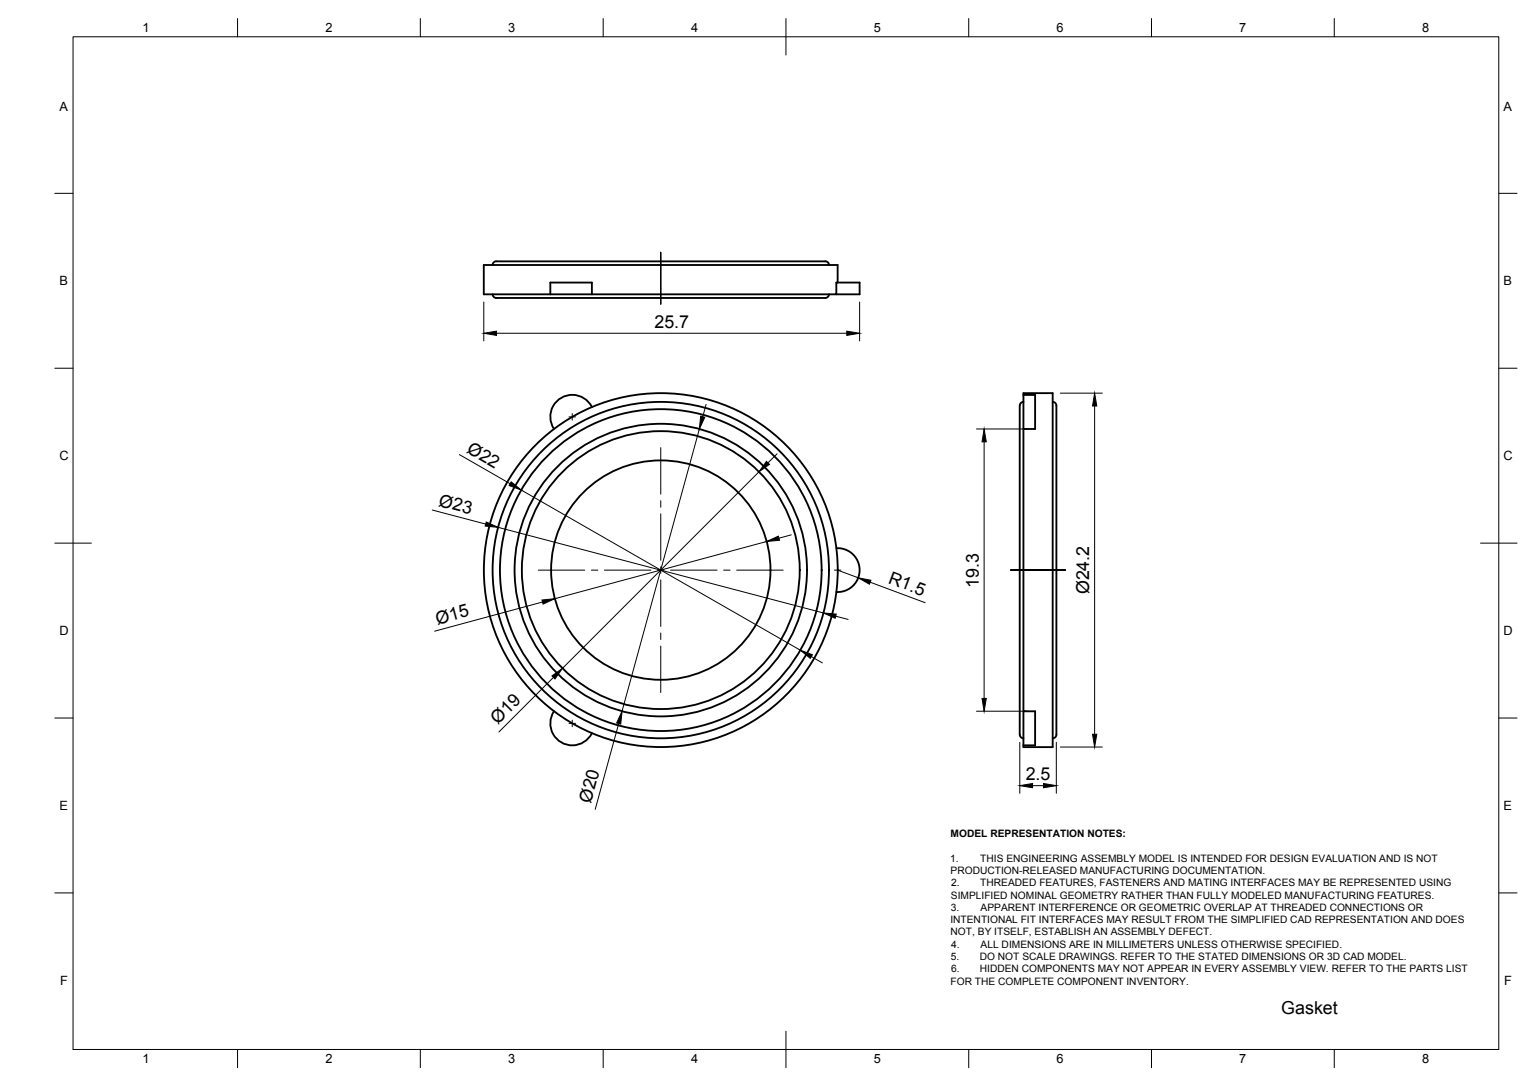
ISO-10303-21;
HEADER;
/* Generated by software containing ST-Developer
 * from STEP Tools, Inc. (www.steptools.com) 
 */

FILE_DESCRIPTION(
/* description */ ('STEP AP214'),
/* implementation_level */ '2;1');

FILE_NAME(
/* name */ 'Gasket.step',
/* time_stamp */ '2026-10-05T23:18:41-07:00',
/* author */ (''),
/* organization */ (''),
/* preprocessor_version */ 'ST-DEVELOPER v20.2',
/* originating_system */ 'Autodesk Translation Framework v15.15.0.0',
/* authorisation */ '');

FILE_SCHEMA (('AUTOMOTIVE_DESIGN { 1 0 10303 214 3 1 1 }'));
ENDSEC;

DATA;
#10=MECHANICAL_DESIGN_GEOMETRIC_PRESENTATION_REPRESENTATION('',(#105),#221662);
#67=MANIFOLD_SOLID_BREP('Body1',#79327);
#79=SHAPE_REPRESENTATION_RELATIONSHIP('SRR','None',#221714,#92);
#92=ADVANCED_BREP_SHAPE_REPRESENTATION('',(#67),#221654);
#105=STYLED_ITEM('',(#221783),#67);
#291=FACE_BOUND('',#24797,.T.);
#292=FACE_BOUND('',#24799,.T.);
#293=FACE_BOUND('',#24801,.T.);
#294=FACE_BOUND('',#24803,.T.);
#295=FACE_BOUND('',#24805,.T.);
#296=FACE_BOUND('',#24807,.T.);
#1892=TOROIDAL_SURFACE('',#80720,9.75,0.25);
#1893=TOROIDAL_SURFACE('',#80724,11.25,0.25);
#1894=TOROIDAL_SURFACE('',#80737,11.25,0.25);
#1895=TOROIDAL_SURFACE('',#80741,9.75,0.25);
#2228=CYLINDRICAL_SURFACE('',#80728,12.1);
#2229=CYLINDRICAL_SURFACE('',#80745,7.50000000000001);
#2230=CYLINDRICAL_SURFACE('',#80748,1.5);
#2231=CYLINDRICAL_SURFACE('',#80751,1.5);
#2232=CYLINDRICAL_SURFACE('',#80757,1.5);
#3145=LINE('',#177883,#10212);
#3146=LINE('',#177887,#10213);
#3147=LINE('',#177891,#10214);
#3148=LINE('',#177895,#10215);
#3149=LINE('',#177899,#10216);
#3150=LINE('',#177903,#10217);
#3151=LINE('',#177907,#10218);
#3152=LINE('',#177925,#10219);
#10212=VECTOR('',#89104,12.1);
#10213=VECTOR('',#89107,1000.);
#10214=VECTOR('',#89110,1000.);
#10215=VECTOR('',#89113,1000.);
#10216=VECTOR('',#89116,1000.);
#10217=VECTOR('',#89119,1000.);
#10218=VECTOR('',#89122,1000.);
#10219=VECTOR('',#89145,7.50000000000001);
#16980=PLANE('',#80754);
#16981=PLANE('',#80755);
#16982=PLANE('',#80759);
#16983=PLANE('',#80760);
#16984=PLANE('',#80761);
#16985=PLANE('',#80762);
#16986=PLANE('',#80763);
#16987=PLANE('',#80764);
#16988=PLANE('',#80765);
#20723=FACE_OUTER_BOUND('',#24784,.T.);
#20724=FACE_OUTER_BOUND('',#24785,.T.);
#20725=FACE_OUTER_BOUND('',#24786,.T.);
#20726=FACE_OUTER_BOUND('',#24787,.T.);
#20727=FACE_OUTER_BOUND('',#24788,.T.);
#20728=FACE_OUTER_BOUND('',#24789,.T.);
#20729=FACE_OUTER_BOUND('',#24790,.T.);
#20730=FACE_OUTER_BOUND('',#24791,.T.);
#20731=FACE_OUTER_BOUND('',#24792,.T.);
#20732=FACE_OUTER_BOUND('',#24793,.T.);
#20733=FACE_OUTER_BOUND('',#24794,.T.);
#20734=FACE_OUTER_BOUND('',#24795,.T.);
#20735=FACE_OUTER_BOUND('',#24796,.T.);
#20736=FACE_OUTER_BOUND('',#24798,.T.);
#20737=FACE_OUTER_BOUND('',#24800,.T.);
#20738=FACE_OUTER_BOUND('',#24802,.T.);
#20739=FACE_OUTER_BOUND('',#24804,.T.);
#20740=FACE_OUTER_BOUND('',#24806,.T.);
#24784=EDGE_LOOP('',(#56581,#56582,#56583,#56584));
#24785=EDGE_LOOP('',(#56585,#56586,#56587,#56588));
#24786=EDGE_LOOP('',(#56589,#56590,#56591,#56592,#56593,#56594,#56595,#56596,
#56597,#56598,#56599,#56600,#56601,#56602,#56603,#56604));
#24787=EDGE_LOOP('',(#56605,#56606,#56607,#56608));
#24788=EDGE_LOOP('',(#56609,#56610,#56611,#56612));
#24789=EDGE_LOOP('',(#56613,#56614,#56615,#56616));
#24790=EDGE_LOOP('',(#56617,#56618,#56619,#56620));
#24791=EDGE_LOOP('',(#56621,#56622,#56623,#56624));
#24792=EDGE_LOOP('',(#56625,#56626));
#24793=EDGE_LOOP('',(#56627,#56628));
#24794=EDGE_LOOP('',(#56629,#56630,#56631,#56632));
#24795=EDGE_LOOP('',(#56633,#56634));
#24796=EDGE_LOOP('',(#56635));
#24797=EDGE_LOOP('',(#56636));
#24798=EDGE_LOOP('',(#56637));
#24799=EDGE_LOOP('',(#56638));
#24800=EDGE_LOOP('',(#56639));
#24801=EDGE_LOOP('',(#56640));
#24802=EDGE_LOOP('',(#56641,#56642,#56643,#56644,#56645,#56646,#56647));
#24803=EDGE_LOOP('',(#56648));
#24804=EDGE_LOOP('',(#56649));
#24805=EDGE_LOOP('',(#56650));
#24806=EDGE_LOOP('',(#56651));
#24807=EDGE_LOOP('',(#56652));
#31271=CIRCLE('',#80721,9.49999999999999);
#31272=CIRCLE('',#80722,0.25);
#31273=CIRCLE('',#80723,10.);
#31274=CIRCLE('',#80725,11.);
#31275=CIRCLE('',#80726,0.25);
#31276=CIRCLE('',#80727,11.5);
#31277=CIRCLE('',#80729,12.1);
#31278=CIRCLE('',#80730,12.1);
#31279=CIRCLE('',#80731,12.1);
#31280=CIRCLE('',#80732,12.1);
#31281=CIRCLE('',#80733,12.1);
#31282=CIRCLE('',#80734,12.1);
#31283=CIRCLE('',#80735,12.1);
#31284=CIRCLE('',#80736,12.1);
#31285=CIRCLE('',#80738,11.5);
#31286=CIRCLE('',#80739,0.25);
#31287=CIRCLE('',#80740,11.);
#31288=CIRCLE('',#80742,10.);
#31289=CIRCLE('',#80743,0.25);
#31290=CIRCLE('',#80744,9.49999999999999);
#31291=CIRCLE('',#80746,7.50000000000001);
#31292=CIRCLE('',#80747,7.50000000000001);
#31293=CIRCLE('',#80749,1.5);
#31294=CIRCLE('',#80750,1.5);
#31295=CIRCLE('',#80752,1.49999999999999);
#31296=CIRCLE('',#80753,1.49999999999999);
#31297=CIRCLE('',#80756,1.5);
#31298=CIRCLE('',#80758,1.5);
#34834=VERTEX_POINT('',#177868);
#34835=VERTEX_POINT('',#177870);
#34836=VERTEX_POINT('',#177874);
#34837=VERTEX_POINT('',#177876);
#34838=VERTEX_POINT('',#177880);
#34839=VERTEX_POINT('',#177882);
#34840=VERTEX_POINT('',#177884);
#34841=VERTEX_POINT('',#177886);
#34842=VERTEX_POINT('',#177888);
#34843=VERTEX_POINT('',#177890);
#34844=VERTEX_POINT('',#177892);
#34845=VERTEX_POINT('',#177894);
#34846=VERTEX_POINT('',#177896);
#34847=VERTEX_POINT('',#177898);
#34848=VERTEX_POINT('',#177900);
#34849=VERTEX_POINT('',#177902);
#34850=VERTEX_POINT('',#177904);
#34851=VERTEX_POINT('',#177906);
#34852=VERTEX_POINT('',#177910);
#34853=VERTEX_POINT('',#177912);
#34854=VERTEX_POINT('',#177916);
#34855=VERTEX_POINT('',#177918);
#34856=VERTEX_POINT('',#177922);
#34857=VERTEX_POINT('',#177924);
#43123=EDGE_CURVE('',#34834,#34834,#31271,.T.);
#43124=EDGE_CURVE('',#34834,#34835,#31272,.T.);
#43125=EDGE_CURVE('',#34835,#34835,#31273,.T.);
#43126=EDGE_CURVE('',#34836,#34836,#31274,.T.);
#43127=EDGE_CURVE('',#34836,#34837,#31275,.T.);
#43128=EDGE_CURVE('',#34837,#34837,#31276,.T.);
#43129=EDGE_CURVE('',#34838,#34838,#31277,.T.);
#43130=EDGE_CURVE('',#34838,#34839,#3145,.T.);
#43131=EDGE_CURVE('',#34839,#34840,#31278,.T.);
#43132=EDGE_CURVE('',#34841,#34840,#3146,.T.);
#43133=EDGE_CURVE('',#34841,#34842,#31279,.T.);
#43134=EDGE_CURVE('',#34843,#34842,#3147,.T.);
#43135=EDGE_CURVE('',#34843,#34844,#31280,.T.);
#43136=EDGE_CURVE('',#34845,#34844,#3148,.T.);
#43137=EDGE_CURVE('',#34845,#34846,#31281,.T.);
#43138=EDGE_CURVE('',#34847,#34846,#3149,.T.);
#43139=EDGE_CURVE('',#34847,#34848,#31282,.T.);
#43140=EDGE_CURVE('',#34849,#34848,#3150,.T.);
#43141=EDGE_CURVE('',#34849,#34850,#31283,.T.);
#43142=EDGE_CURVE('',#34851,#34850,#3151,.T.);
#43143=EDGE_CURVE('',#34851,#34839,#31284,.T.);
#43144=EDGE_CURVE('',#34852,#34852,#31285,.T.);
#43145=EDGE_CURVE('',#34852,#34853,#31286,.T.);
#43146=EDGE_CURVE('',#34853,#34853,#31287,.T.);
#43147=EDGE_CURVE('',#34854,#34854,#31288,.T.);
#43148=EDGE_CURVE('',#34854,#34855,#31289,.T.);
#43149=EDGE_CURVE('',#34855,#34855,#31290,.T.);
#43150=EDGE_CURVE('',#34856,#34856,#31291,.T.);
#43151=EDGE_CURVE('',#34856,#34857,#3152,.T.);
#43152=EDGE_CURVE('',#34857,#34857,#31292,.T.);
#43153=EDGE_CURVE('',#34850,#34849,#31293,.T.);
#43154=EDGE_CURVE('',#34851,#34848,#31294,.T.);
#43155=EDGE_CURVE('',#34842,#34841,#31295,.T.);
#43156=EDGE_CURVE('',#34843,#34840,#31296,.T.);
#43157=EDGE_CURVE('',#34846,#34845,#31297,.T.);
#43158=EDGE_CURVE('',#34847,#34844,#31298,.T.);
#56581=ORIENTED_EDGE('',*,*,#43123,.F.);
#56582=ORIENTED_EDGE('',*,*,#43124,.T.);
#56583=ORIENTED_EDGE('',*,*,#43125,.T.);
#56584=ORIENTED_EDGE('',*,*,#43124,.F.);
#56585=ORIENTED_EDGE('',*,*,#43126,.F.);
#56586=ORIENTED_EDGE('',*,*,#43127,.T.);
#56587=ORIENTED_EDGE('',*,*,#43128,.T.);
#56588=ORIENTED_EDGE('',*,*,#43127,.F.);
#56589=ORIENTED_EDGE('',*,*,#43129,.F.);
#56590=ORIENTED_EDGE('',*,*,#43130,.T.);
#56591=ORIENTED_EDGE('',*,*,#43131,.T.);
#56592=ORIENTED_EDGE('',*,*,#43132,.F.);
#56593=ORIENTED_EDGE('',*,*,#43133,.T.);
#56594=ORIENTED_EDGE('',*,*,#43134,.F.);
#56595=ORIENTED_EDGE('',*,*,#43135,.T.);
#56596=ORIENTED_EDGE('',*,*,#43136,.F.);
#56597=ORIENTED_EDGE('',*,*,#43137,.T.);
#56598=ORIENTED_EDGE('',*,*,#43138,.F.);
#56599=ORIENTED_EDGE('',*,*,#43139,.T.);
#56600=ORIENTED_EDGE('',*,*,#43140,.F.);
#56601=ORIENTED_EDGE('',*,*,#43141,.T.);
#56602=ORIENTED_EDGE('',*,*,#43142,.F.);
#56603=ORIENTED_EDGE('',*,*,#43143,.T.);
#56604=ORIENTED_EDGE('',*,*,#43130,.F.);
#56605=ORIENTED_EDGE('',*,*,#43144,.F.);
#56606=ORIENTED_EDGE('',*,*,#43145,.T.);
#56607=ORIENTED_EDGE('',*,*,#43146,.T.);
#56608=ORIENTED_EDGE('',*,*,#43145,.F.);
#56609=ORIENTED_EDGE('',*,*,#43147,.F.);
#56610=ORIENTED_EDGE('',*,*,#43148,.T.);
#56611=ORIENTED_EDGE('',*,*,#43149,.T.);
#56612=ORIENTED_EDGE('',*,*,#43148,.F.);
#56613=ORIENTED_EDGE('',*,*,#43150,.F.);
#56614=ORIENTED_EDGE('',*,*,#43151,.T.);
#56615=ORIENTED_EDGE('',*,*,#43152,.T.);
#56616=ORIENTED_EDGE('',*,*,#43151,.F.);
#56617=ORIENTED_EDGE('',*,*,#43153,.T.);
#56618=ORIENTED_EDGE('',*,*,#43140,.T.);
#56619=ORIENTED_EDGE('',*,*,#43154,.F.);
#56620=ORIENTED_EDGE('',*,*,#43142,.T.);
#56621=ORIENTED_EDGE('',*,*,#43155,.T.);
#56622=ORIENTED_EDGE('',*,*,#43132,.T.);
#56623=ORIENTED_EDGE('',*,*,#43156,.F.);
#56624=ORIENTED_EDGE('',*,*,#43134,.T.);
#56625=ORIENTED_EDGE('',*,*,#43133,.F.);
#56626=ORIENTED_EDGE('',*,*,#43155,.F.);
#56627=ORIENTED_EDGE('',*,*,#43137,.F.);
#56628=ORIENTED_EDGE('',*,*,#43157,.F.);
#56629=ORIENTED_EDGE('',*,*,#43158,.F.);
#56630=ORIENTED_EDGE('',*,*,#43138,.T.);
#56631=ORIENTED_EDGE('',*,*,#43157,.T.);
#56632=ORIENTED_EDGE('',*,*,#43136,.T.);
#56633=ORIENTED_EDGE('',*,*,#43141,.F.);
#56634=ORIENTED_EDGE('',*,*,#43153,.F.);
#56635=ORIENTED_EDGE('',*,*,#43123,.T.);
#56636=ORIENTED_EDGE('',*,*,#43152,.F.);
#56637=ORIENTED_EDGE('',*,*,#43149,.F.);
#56638=ORIENTED_EDGE('',*,*,#43150,.T.);
#56639=ORIENTED_EDGE('',*,*,#43146,.F.);
#56640=ORIENTED_EDGE('',*,*,#43147,.T.);
#56641=ORIENTED_EDGE('',*,*,#43135,.F.);
#56642=ORIENTED_EDGE('',*,*,#43156,.T.);
#56643=ORIENTED_EDGE('',*,*,#43131,.F.);
#56644=ORIENTED_EDGE('',*,*,#43143,.F.);
#56645=ORIENTED_EDGE('',*,*,#43154,.T.);
#56646=ORIENTED_EDGE('',*,*,#43139,.F.);
#56647=ORIENTED_EDGE('',*,*,#43158,.T.);
#56648=ORIENTED_EDGE('',*,*,#43144,.T.);
#56649=ORIENTED_EDGE('',*,*,#43129,.T.);
#56650=ORIENTED_EDGE('',*,*,#43128,.F.);
#56651=ORIENTED_EDGE('',*,*,#43126,.T.);
#56652=ORIENTED_EDGE('',*,*,#43125,.F.);
#76153=ADVANCED_FACE('',(#20723),#1892,.T.);
#76154=ADVANCED_FACE('',(#20724),#1893,.T.);
#76155=ADVANCED_FACE('',(#20725),#2228,.T.);
#76156=ADVANCED_FACE('',(#20726),#1894,.T.);
#76157=ADVANCED_FACE('',(#20727),#1895,.T.);
#76158=ADVANCED_FACE('',(#20728),#2229,.F.);
#76159=ADVANCED_FACE('',(#20729),#2230,.T.);
#76160=ADVANCED_FACE('',(#20730),#2231,.T.);
#76161=ADVANCED_FACE('',(#20731),#16980,.F.);
#76162=ADVANCED_FACE('',(#20732),#16981,.F.);
#76163=ADVANCED_FACE('',(#20733),#2232,.T.);
#76164=ADVANCED_FACE('',(#20734),#16982,.F.);
#76165=ADVANCED_FACE('',(#20735,#291),#16983,.T.);
#76166=ADVANCED_FACE('',(#20736,#292),#16984,.T.);
#76167=ADVANCED_FACE('',(#20737,#293),#16985,.T.);
#76168=ADVANCED_FACE('',(#20738,#294),#16986,.T.);
#76169=ADVANCED_FACE('',(#20739,#295),#16987,.T.);
#76170=ADVANCED_FACE('',(#20740,#296),#16988,.T.);
#79327=CLOSED_SHELL('',(#76153,#76154,#76155,#76156,#76157,#76158,#76159,
#76160,#76161,#76162,#76163,#76164,#76165,#76166,#76167,#76168,#76169,#76170));
#80719=AXIS2_PLACEMENT_3D('',#177866,#89082,#89083);
#80720=AXIS2_PLACEMENT_3D('',#177867,#89084,#89085);
#80721=AXIS2_PLACEMENT_3D('',#177869,#89086,#89087);
#80722=AXIS2_PLACEMENT_3D('',#177871,#89088,#89089);
#80723=AXIS2_PLACEMENT_3D('',#177872,#89090,#89091);
#80724=AXIS2_PLACEMENT_3D('',#177873,#89092,#89093);
#80725=AXIS2_PLACEMENT_3D('',#177875,#89094,#89095);
#80726=AXIS2_PLACEMENT_3D('',#177877,#89096,#89097);
#80727=AXIS2_PLACEMENT_3D('',#177878,#89098,#89099);
#80728=AXIS2_PLACEMENT_3D('',#177879,#89100,#89101);
#80729=AXIS2_PLACEMENT_3D('',#177881,#89102,#89103);
#80730=AXIS2_PLACEMENT_3D('',#177885,#89105,#89106);
#80731=AXIS2_PLACEMENT_3D('',#177889,#89108,#89109);
#80732=AXIS2_PLACEMENT_3D('',#177893,#89111,#89112);
#80733=AXIS2_PLACEMENT_3D('',#177897,#89114,#89115);
#80734=AXIS2_PLACEMENT_3D('',#177901,#89117,#89118);
#80735=AXIS2_PLACEMENT_3D('',#177905,#89120,#89121);
#80736=AXIS2_PLACEMENT_3D('',#177908,#89123,#89124);
#80737=AXIS2_PLACEMENT_3D('',#177909,#89125,#89126);
#80738=AXIS2_PLACEMENT_3D('',#177911,#89127,#89128);
#80739=AXIS2_PLACEMENT_3D('',#177913,#89129,#89130);
#80740=AXIS2_PLACEMENT_3D('',#177914,#89131,#89132);
#80741=AXIS2_PLACEMENT_3D('',#177915,#89133,#89134);
#80742=AXIS2_PLACEMENT_3D('',#177917,#89135,#89136);
#80743=AXIS2_PLACEMENT_3D('',#177919,#89137,#89138);
#80744=AXIS2_PLACEMENT_3D('',#177920,#89139,#89140);
#80745=AXIS2_PLACEMENT_3D('',#177921,#89141,#89142);
#80746=AXIS2_PLACEMENT_3D('',#177923,#89143,#89144);
#80747=AXIS2_PLACEMENT_3D('',#177926,#89146,#89147);
#80748=AXIS2_PLACEMENT_3D('',#177927,#89148,#89149);
#80749=AXIS2_PLACEMENT_3D('',#177928,#89150,#89151);
#80750=AXIS2_PLACEMENT_3D('',#177929,#89152,#89153);
#80751=AXIS2_PLACEMENT_3D('',#177930,#89154,#89155);
#80752=AXIS2_PLACEMENT_3D('',#177931,#89156,#89157);
#80753=AXIS2_PLACEMENT_3D('',#177932,#89158,#89159);
#80754=AXIS2_PLACEMENT_3D('',#177933,#89160,#89161);
#80755=AXIS2_PLACEMENT_3D('',#177934,#89162,#89163);
#80756=AXIS2_PLACEMENT_3D('',#177935,#89164,#89165);
#80757=AXIS2_PLACEMENT_3D('',#177936,#89166,#89167);
#80758=AXIS2_PLACEMENT_3D('',#177937,#89168,#89169);
#80759=AXIS2_PLACEMENT_3D('',#177938,#89170,#89171);
#80760=AXIS2_PLACEMENT_3D('',#177939,#89172,#89173);
#80761=AXIS2_PLACEMENT_3D('',#177940,#89174,#89175);
#80762=AXIS2_PLACEMENT_3D('',#177941,#89176,#89177);
#80763=AXIS2_PLACEMENT_3D('',#177942,#89178,#89179);
#80764=AXIS2_PLACEMENT_3D('',#177943,#89180,#89181);
#80765=AXIS2_PLACEMENT_3D('',#177944,#89182,#89183);
#89082=DIRECTION('axis',(0.,0.,1.));
#89083=DIRECTION('refdir',(1.,0.,0.));
#89084=DIRECTION('center_axis',(1.,0.,0.));
#89085=DIRECTION('ref_axis',(0.,0.,-1.));
#89086=DIRECTION('center_axis',(1.,0.,0.));
#89087=DIRECTION('ref_axis',(0.,0.,-1.));
#89088=DIRECTION('center_axis',(0.,-1.,0.));
#89089=DIRECTION('ref_axis',(0.,0.,1.));
#89090=DIRECTION('center_axis',(1.,0.,0.));
#89091=DIRECTION('ref_axis',(0.,0.,-1.));
#89092=DIRECTION('center_axis',(1.,0.,0.));
#89093=DIRECTION('ref_axis',(0.,0.,-1.));
#89094=DIRECTION('center_axis',(1.,0.,0.));
#89095=DIRECTION('ref_axis',(0.,0.,-1.));
#89096=DIRECTION('center_axis',(0.,-1.,0.));
#89097=DIRECTION('ref_axis',(0.,0.,1.));
#89098=DIRECTION('center_axis',(1.,0.,0.));
#89099=DIRECTION('ref_axis',(0.,0.,-1.));
#89100=DIRECTION('center_axis',(1.,0.,0.));
#89101=DIRECTION('ref_axis',(0.,0.,-1.));
#89102=DIRECTION('center_axis',(1.,0.,0.));
#89103=DIRECTION('ref_axis',(0.,0.,-1.));
#89104=DIRECTION('',(-1.,0.,0.));
#89105=DIRECTION('center_axis',(1.,0.,0.));
#89106=DIRECTION('ref_axis',(0.,0.,-1.));
#89107=DIRECTION('',(-1.,0.,0.));
#89108=DIRECTION('center_axis',(1.,0.,0.));
#89109=DIRECTION('ref_axis',(0.,0.,1.));
#89110=DIRECTION('',(1.,0.,0.));
#89111=DIRECTION('center_axis',(1.,0.,0.));
#89112=DIRECTION('ref_axis',(0.,0.,-1.));
#89113=DIRECTION('',(-1.,0.,0.));
#89114=DIRECTION('center_axis',(1.,0.,0.));
#89115=DIRECTION('ref_axis',(0.,0.,1.));
#89116=DIRECTION('',(1.,0.,0.));
#89117=DIRECTION('center_axis',(1.,0.,0.));
#89118=DIRECTION('ref_axis',(0.,0.,-1.));
#89119=DIRECTION('',(-1.,0.,0.));
#89120=DIRECTION('center_axis',(1.,0.,0.));
#89121=DIRECTION('ref_axis',(0.,0.,1.));
#89122=DIRECTION('',(1.,0.,0.));
#89123=DIRECTION('center_axis',(1.,0.,0.));
#89124=DIRECTION('ref_axis',(0.,0.,-1.));
#89125=DIRECTION('center_axis',(1.,0.,0.));
#89126=DIRECTION('ref_axis',(0.,0.,-1.));
#89127=DIRECTION('center_axis',(1.,0.,0.));
#89128=DIRECTION('ref_axis',(0.,0.,-1.));
#89129=DIRECTION('center_axis',(0.,-1.,0.));
#89130=DIRECTION('ref_axis',(0.,0.,1.));
#89131=DIRECTION('center_axis',(1.,0.,0.));
#89132=DIRECTION('ref_axis',(0.,0.,-1.));
#89133=DIRECTION('center_axis',(1.,0.,0.));
#89134=DIRECTION('ref_axis',(0.,0.,-1.));
#89135=DIRECTION('center_axis',(1.,0.,0.));
#89136=DIRECTION('ref_axis',(0.,0.,-1.));
#89137=DIRECTION('center_axis',(0.,-1.,0.));
#89138=DIRECTION('ref_axis',(0.,0.,1.));
#89139=DIRECTION('center_axis',(1.,0.,0.));
#89140=DIRECTION('ref_axis',(0.,0.,-1.));
#89141=DIRECTION('center_axis',(1.,0.,0.));
#89142=DIRECTION('ref_axis',(0.,0.,-1.));
#89143=DIRECTION('center_axis',(1.,0.,0.));
#89144=DIRECTION('ref_axis',(0.,0.,-1.));
#89145=DIRECTION('',(1.,0.,0.));
#89146=DIRECTION('center_axis',(1.,0.,0.));
#89147=DIRECTION('ref_axis',(0.,0.,-1.));
#89148=DIRECTION('center_axis',(-1.,0.,0.));
#89149=DIRECTION('ref_axis',(0.,1.,-1.71512449944288E-15));
#89150=DIRECTION('center_axis',(-1.,0.,0.));
#89151=DIRECTION('ref_axis',(0.,1.,0.));
#89152=DIRECTION('center_axis',(-1.,0.,0.));
#89153=DIRECTION('ref_axis',(0.,1.,0.));
#89154=DIRECTION('center_axis',(-1.,0.,0.));
#89155=DIRECTION('ref_axis',(0.,0.,1.));
#89156=DIRECTION('center_axis',(-1.,0.,0.));
#89157=DIRECTION('ref_axis',(0.,-0.500000000000002,0.866025403784437));
#89158=DIRECTION('center_axis',(-1.,0.,0.));
#89159=DIRECTION('ref_axis',(0.,-0.500000000000002,0.866025403784437));
#89160=DIRECTION('center_axis',(-1.,0.,0.));
#89161=DIRECTION('ref_axis',(0.,0.,1.));
#89162=DIRECTION('center_axis',(-1.,0.,0.));
#89163=DIRECTION('ref_axis',(0.,0.,1.));
#89164=DIRECTION('center_axis',(-1.,0.,0.));
#89165=DIRECTION('ref_axis',(0.,-0.500000000000001,-0.866025403784438));
#89166=DIRECTION('center_axis',(-1.,0.,0.));
#89167=DIRECTION('ref_axis',(0.,-0.499999999999999,-0.866025403784439));
#89168=DIRECTION('center_axis',(-1.,0.,0.));
#89169=DIRECTION('ref_axis',(0.,-0.500000000000001,-0.866025403784438));
#89170=DIRECTION('center_axis',(-1.,0.,0.));
#89171=DIRECTION('ref_axis',(0.,0.,1.));
#89172=DIRECTION('center_axis',(1.,0.,0.));
#89173=DIRECTION('ref_axis',(0.,1.,0.));
#89174=DIRECTION('center_axis',(-1.,0.,0.));
#89175=DIRECTION('ref_axis',(0.,0.,1.));
#89176=DIRECTION('center_axis',(-1.,0.,0.));
#89177=DIRECTION('ref_axis',(0.,0.,1.));
#89178=DIRECTION('center_axis',(-1.,0.,0.));
#89179=DIRECTION('ref_axis',(0.,0.,1.));
#89180=DIRECTION('center_axis',(1.,0.,0.));
#89181=DIRECTION('ref_axis',(0.,1.,0.));
#89182=DIRECTION('center_axis',(1.,0.,0.));
#89183=DIRECTION('ref_axis',(0.,1.,0.));
#177866=CARTESIAN_POINT('',(0.,0.,0.));
#177867=CARTESIAN_POINT('Origin',(-20.5675364832709,75.,72.98888938658));
#177868=CARTESIAN_POINT('',(-20.5675364832709,75.,82.48888938658));
#177869=CARTESIAN_POINT('Origin',(-20.5675364832709,75.,72.98888938658));
#177870=CARTESIAN_POINT('',(-20.5675364832709,75.,82.98888938658));
#177871=CARTESIAN_POINT('Origin',(-20.5675364832709,75.,82.73888938658));
#177872=CARTESIAN_POINT('Origin',(-20.5675364832709,75.,72.98888938658));
#177873=CARTESIAN_POINT('Origin',(-20.5675364832709,75.,72.98888938658));
#177874=CARTESIAN_POINT('',(-20.5675364832709,75.,83.98888938658));
#177875=CARTESIAN_POINT('Origin',(-20.5675364832709,75.,72.98888938658));
#177876=CARTESIAN_POINT('',(-20.5675364832709,75.,84.48888938658));
#177877=CARTESIAN_POINT('Origin',(-20.5675364832709,75.,84.23888938658));
#177878=CARTESIAN_POINT('Origin',(-20.5675364832709,75.,72.98888938658));
#177879=CARTESIAN_POINT('Origin',(-25.5675364832709,75.,72.98888938658));
#177880=CARTESIAN_POINT('',(-20.5675364832709,75.,85.08888938658));
#177881=CARTESIAN_POINT('Origin',(-20.5675364832709,75.,72.98888938658));
#177882=CARTESIAN_POINT('',(-22.5675364832709,75.,85.08888938658));
#177883=CARTESIAN_POINT('',(-25.5675364832709,75.,85.08888938658));
#177884=CARTESIAN_POINT('',(-22.5675364832709,70.2930278873758,84.1358357635471));
#177885=CARTESIAN_POINT('Origin',(-22.5675364832709,75.,72.98888938658));
#177886=CARTESIAN_POINT('',(-21.7675364832709,70.2930278873758,84.1358357635471));
#177887=CARTESIAN_POINT('',(-22.1675364832709,70.2930278873758,84.1358357635471));
#177888=CARTESIAN_POINT('',(-21.7675364832709,67.6999473192355,82.6387199995009));
#177889=CARTESIAN_POINT('Origin',(-21.7675364832709,75.,72.98888938658));
#177890=CARTESIAN_POINT('',(-22.5675364832709,67.6999473192355,82.6387199995009));
#177891=CARTESIAN_POINT('',(-22.1675364832709,67.6999473192355,82.6387199995009));
#177892=CARTESIAN_POINT('',(-22.5675364832709,67.6999473192356,63.3390587736591));
#177893=CARTESIAN_POINT('Origin',(-22.5675364832709,75.,72.98888938658));
#177894=CARTESIAN_POINT('',(-21.7675364832709,67.6999473192356,63.3390587736591));
#177895=CARTESIAN_POINT('',(-22.1675364832709,67.6999473192356,63.3390587736591));
#177896=CARTESIAN_POINT('',(-21.7675364832709,70.2930278873759,61.8419430096129));
#177897=CARTESIAN_POINT('Origin',(-21.7675364832709,75.,72.98888938658));
#177898=CARTESIAN_POINT('',(-22.5675364832709,70.2930278873759,61.8419430096129));
#177899=CARTESIAN_POINT('',(-22.1675364832709,70.2930278873759,61.8419430096129));
#177900=CARTESIAN_POINT('',(-22.5675364832709,87.0070247933884,71.4917736225339));
#177901=CARTESIAN_POINT('Origin',(-22.5675364832709,75.,72.98888938658));
#177902=CARTESIAN_POINT('',(-21.7675364832709,87.0070247933884,71.4917736225339));
#177903=CARTESIAN_POINT('',(-22.1675364832709,87.0070247933884,71.4917736225339));
#177904=CARTESIAN_POINT('',(-21.7675364832709,87.0070247933884,74.4860051506262));
#177905=CARTESIAN_POINT('Origin',(-21.7675364832709,75.,72.98888938658));
#177906=CARTESIAN_POINT('',(-22.5675364832709,87.0070247933884,74.4860051506262));
#177907=CARTESIAN_POINT('',(-22.1675364832709,87.0070247933884,74.4860051506262));
#177908=CARTESIAN_POINT('Origin',(-22.5675364832709,75.,72.98888938658));
#177909=CARTESIAN_POINT('Origin',(-22.5675364832709,75.,72.98888938658));
#177910=CARTESIAN_POINT('',(-22.5675364832709,75.,84.48888938658));
#177911=CARTESIAN_POINT('Origin',(-22.5675364832709,75.,72.98888938658));
#177912=CARTESIAN_POINT('',(-22.5675364832709,75.,83.98888938658));
#177913=CARTESIAN_POINT('Origin',(-22.5675364832709,75.,84.23888938658));
#177914=CARTESIAN_POINT('Origin',(-22.5675364832709,75.,72.98888938658));
#177915=CARTESIAN_POINT('Origin',(-22.5675364832709,75.,72.98888938658));
#177916=CARTESIAN_POINT('',(-22.5675364832709,75.,82.98888938658));
#177917=CARTESIAN_POINT('Origin',(-22.5675364832709,75.,72.98888938658));
#177918=CARTESIAN_POINT('',(-22.5675364832709,75.,82.48888938658));
#177919=CARTESIAN_POINT('Origin',(-22.5675364832709,75.,82.73888938658));
#177920=CARTESIAN_POINT('Origin',(-22.5675364832709,75.,72.98888938658));
#177921=CARTESIAN_POINT('Origin',(-25.5675364832709,75.,72.98888938658));
#177922=CARTESIAN_POINT('',(-22.5675364832709,75.,80.48888938658));
#177923=CARTESIAN_POINT('Origin',(-22.5675364832709,75.,72.98888938658));
#177924=CARTESIAN_POINT('',(-20.5675364832709,75.,80.48888938658));
#177925=CARTESIAN_POINT('',(-25.5675364832709,75.,80.48888938658));
#177926=CARTESIAN_POINT('Origin',(-20.5675364832709,75.,72.98888938658));
#177927=CARTESIAN_POINT('Origin',(-21.7675364832709,87.1,72.98888938658));
#177928=CARTESIAN_POINT('Origin',(-21.7675364832709,87.1,72.98888938658));
#177929=CARTESIAN_POINT('Origin',(-22.5675364832709,87.1,72.98888938658));
#177930=CARTESIAN_POINT('Origin',(-21.7675364832709,68.95,83.4677967723717));
#177931=CARTESIAN_POINT('Origin',(-21.7675364832709,68.95,83.4677967723717));
#177932=CARTESIAN_POINT('Origin',(-22.5675364832709,68.95,83.4677967723717));
#177933=CARTESIAN_POINT('Origin',(-21.7675364832709,68.95,83.4677967723717));
#177934=CARTESIAN_POINT('Origin',(-21.7675364832709,68.95,62.5099820007883));
#177935=CARTESIAN_POINT('Origin',(-21.7675364832709,68.95,62.5099820007883));
#177936=CARTESIAN_POINT('Origin',(-21.7675364832709,68.95,62.5099820007883));
#177937=CARTESIAN_POINT('Origin',(-22.5675364832709,68.95,62.5099820007883));
#177938=CARTESIAN_POINT('Origin',(-21.7675364832709,87.1,72.98888938658));
#177939=CARTESIAN_POINT('Origin',(-20.5675364832709,67.5,72.98888938658));
#177940=CARTESIAN_POINT('Origin',(-22.5675364832709,65.5,72.98888938658));
#177941=CARTESIAN_POINT('Origin',(-22.5675364832709,64.,72.98888938658));
#177942=CARTESIAN_POINT('Origin',(-22.5675364832709,62.9,72.98888938658));
#177943=CARTESIAN_POINT('Origin',(-20.5675364832709,63.5,72.98888938658));
#177944=CARTESIAN_POINT('Origin',(-20.5675364832709,65.,72.98888938658));
#221639=UNCERTAINTY_MEASURE_WITH_UNIT(LENGTH_MEASURE(0.01),#221663,
'DISTANCE_ACCURACY_VALUE',
'Maximum model space distance between geometric entities at asserted c
onnectivities');
#221647=UNCERTAINTY_MEASURE_WITH_UNIT(LENGTH_MEASURE(0.01),#221663,
'DISTANCE_ACCURACY_VALUE',
'Maximum model space distance between geometric entities at asserted c
onnectivities');
#221654=(
GEOMETRIC_REPRESENTATION_CONTEXT(3)
GLOBAL_UNCERTAINTY_ASSIGNED_CONTEXT((#221639))
GLOBAL_UNIT_ASSIGNED_CONTEXT((#221663,#221665,#221666))
REPRESENTATION_CONTEXT('','3D')
);
#221662=(
GEOMETRIC_REPRESENTATION_CONTEXT(3)
GLOBAL_UNCERTAINTY_ASSIGNED_CONTEXT((#221647))
GLOBAL_UNIT_ASSIGNED_CONTEXT((#221663,#221665,#221666))
REPRESENTATION_CONTEXT('','3D')
);
#221663=(
LENGTH_UNIT()
NAMED_UNIT(*)
SI_UNIT(.MILLI.,.METRE.)
);
#221665=(
NAMED_UNIT(*)
PLANE_ANGLE_UNIT()
SI_UNIT($,.RADIAN.)
);
#221666=(
NAMED_UNIT(*)
SI_UNIT($,.STERADIAN.)
SOLID_ANGLE_UNIT()
);
#221673=SHAPE_DEFINITION_REPRESENTATION(#221687,#221714);
#221687=PRODUCT_DEFINITION_SHAPE('',$,#221729);
#221714=SHAPE_REPRESENTATION('',(#80719),#221654);
#221722=PRODUCT_DEFINITION_CONTEXT('part definition',#221766,'design');
#221729=PRODUCT_DEFINITION('2026-10-05-23-02-36-870','Gasket',#221743,#221722);
#221743=PRODUCT_DEFINITION_FORMATION('',$,#221774);
#221766=APPLICATION_CONTEXT(
'Core Data for Automotive Mechanical Design Process');
#221767=PRODUCT_CONTEXT('part definition',#221766,'mechanical');
#221774=PRODUCT('2026-10-05-23-02-36-870','Gasket',$,(#221767));
#221783=PRESENTATION_STYLE_ASSIGNMENT((#221785));
#221785=SURFACE_STYLE_USAGE(.BOTH.,#221787);
#221787=SURFACE_SIDE_STYLE('',(#221789));
#221789=SURFACE_STYLE_FILL_AREA(#221791);
#221791=FILL_AREA_STYLE('Opaque(202,209,238)',(#221793));
#221793=FILL_AREA_STYLE_COLOUR('Opaque(202,209,238)',#221795);
#221795=COLOUR_RGB('Opaque(202,209,238)', 0.09019608, 0.27058824, 0.51372549);
ENDSEC;
END-ISO-10303-21;
